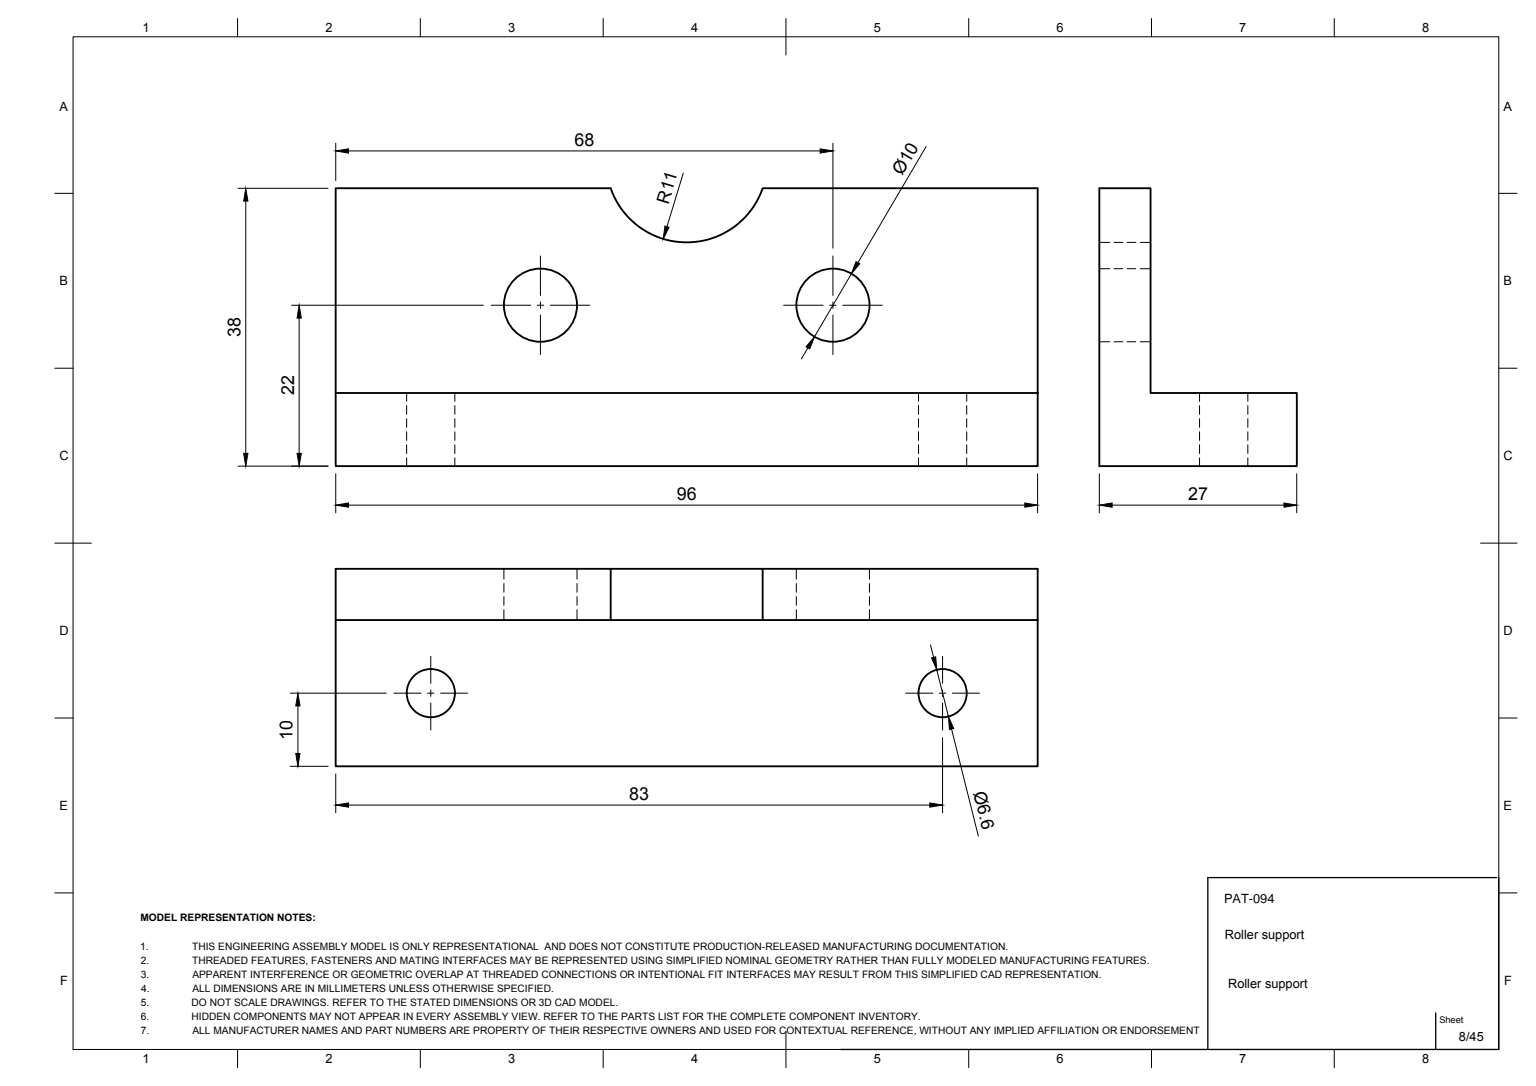
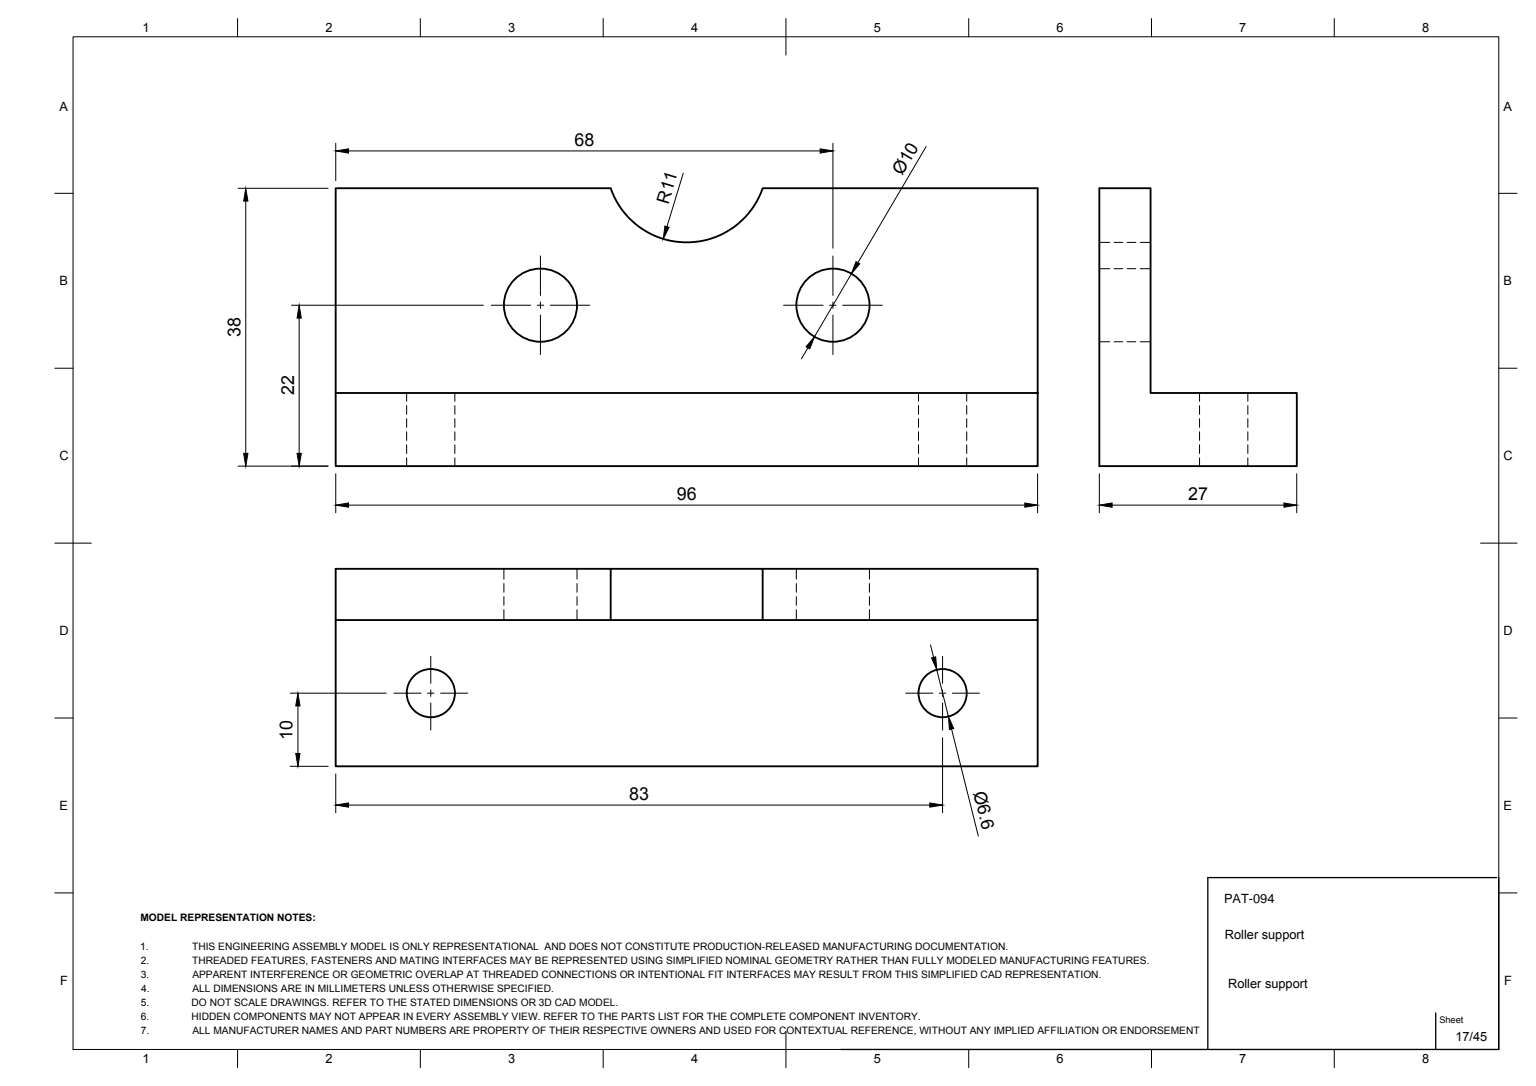
ISO-10303-21;
HEADER;
/* Generated by software containing ST-Developer
 * from STEP Tools, Inc. (www.steptools.com) 
 */

FILE_DESCRIPTION(
/* description */ ('Shaft runout checking stand'),
/* implementation_level */ '2;1');

FILE_NAME(
/* name */ 'Roller support.step',
/* time_stamp */ '2026-11-02T21:12:33-08:00',
/* author */ (''),
/* organization */ (''),
/* preprocessor_version */ 'ST-DEVELOPER v20.2',
/* originating_system */ 'Autodesk Translation Framework v15.17.0.0',
/* authorisation */ '');

FILE_SCHEMA (('AUTOMOTIVE_DESIGN { 1 0 10303 214 3 1 1 }'));
ENDSEC;

DATA;
#10=MECHANICAL_DESIGN_GEOMETRIC_PRESENTATION_REPRESENTATION('',(#469),#11748);
#383=SHAPE_REPRESENTATION_RELATIONSHIP('SRR','None',#11932,#426);
#426=ADVANCED_BREP_SHAPE_REPRESENTATION('',(#520),#11708);
#469=STYLED_ITEM('',(#12169),#520);
#520=MANIFOLD_SOLID_BREP('Body1',#6212);
#591=FACE_BOUND('',#1535,.T.);
#592=FACE_BOUND('',#1536,.T.);
#593=FACE_BOUND('',#1541,.T.);
#594=FACE_BOUND('',#1542,.T.);
#595=FACE_BOUND('',#1546,.T.);
#596=FACE_BOUND('',#1547,.T.);
#597=FACE_BOUND('',#1551,.T.);
#598=FACE_BOUND('',#1552,.T.);
#708=CIRCLE('',#6877,0.33);
#709=CIRCLE('',#6878,0.33);
#710=CIRCLE('',#6880,0.33);
#711=CIRCLE('',#6881,0.33);
#712=CIRCLE('',#6883,1.1);
#713=CIRCLE('',#6884,1.1);
#714=CIRCLE('',#6886,0.5);
#715=CIRCLE('',#6887,0.5);
#716=CIRCLE('',#6890,0.5);
#717=CIRCLE('',#6892,0.5);
#954=CYLINDRICAL_SURFACE('',#6876,0.33);
#955=CYLINDRICAL_SURFACE('',#6879,0.33);
#956=CYLINDRICAL_SURFACE('',#6882,1.1);
#957=CYLINDRICAL_SURFACE('',#6889,0.5);
#958=CYLINDRICAL_SURFACE('',#6891,0.5);
#1134=FACE_OUTER_BOUND('',#1531,.T.);
#1135=FACE_OUTER_BOUND('',#1532,.T.);
#1136=FACE_OUTER_BOUND('',#1533,.T.);
#1137=FACE_OUTER_BOUND('',#1534,.T.);
#1138=FACE_OUTER_BOUND('',#1537,.T.);
#1139=FACE_OUTER_BOUND('',#1538,.T.);
#1140=FACE_OUTER_BOUND('',#1539,.T.);
#1141=FACE_OUTER_BOUND('',#1540,.T.);
#1142=FACE_OUTER_BOUND('',#1543,.T.);
#1143=FACE_OUTER_BOUND('',#1544,.T.);
#1144=FACE_OUTER_BOUND('',#1545,.T.);
#1145=FACE_OUTER_BOUND('',#1548,.T.);
#1146=FACE_OUTER_BOUND('',#1549,.T.);
#1147=FACE_OUTER_BOUND('',#1550,.T.);
#1531=EDGE_LOOP('',(#4596,#4597,#4598,#4599));
#1532=EDGE_LOOP('',(#4600,#4601,#4602,#4603));
#1533=EDGE_LOOP('',(#4604,#4605,#4606,#4607));
#1534=EDGE_LOOP('',(#4608,#4609,#4610,#4611,#4612,#4613));
#1535=EDGE_LOOP('',(#4614));
#1536=EDGE_LOOP('',(#4615));
#1537=EDGE_LOOP('',(#4616,#4617,#4618,#4619));
#1538=EDGE_LOOP('',(#4620,#4621,#4622,#4623));
#1539=EDGE_LOOP('',(#4624,#4625,#4626,#4627));
#1540=EDGE_LOOP('',(#4628,#4629,#4630,#4631));
#1541=EDGE_LOOP('',(#4632));
#1542=EDGE_LOOP('',(#4633));
#1543=EDGE_LOOP('',(#4634,#4635,#4636,#4637));
#1544=EDGE_LOOP('',(#4638,#4639,#4640,#4641,#4642,#4643));
#1545=EDGE_LOOP('',(#4644,#4645,#4646,#4647,#4648,#4649));
#1546=EDGE_LOOP('',(#4650));
#1547=EDGE_LOOP('',(#4651));
#1548=EDGE_LOOP('',(#4652,#4653,#4654,#4655,#4656,#4657));
#1549=EDGE_LOOP('',(#4658,#4659,#4660,#4661));
#1550=EDGE_LOOP('',(#4662,#4663,#4664,#4665));
#1551=EDGE_LOOP('',(#4666));
#1552=EDGE_LOOP('',(#4667));
#2102=LINE('',#10007,#2569);
#2103=LINE('',#10013,#2570);
#2104=LINE('',#10020,#2571);
#2105=LINE('',#10023,#2572);
#2106=LINE('',#10026,#2573);
#2107=LINE('',#10028,#2574);
#2108=LINE('',#10030,#2575);
#2109=LINE('',#10032,#2576);
#2110=LINE('',#10033,#2577);
#2111=LINE('',#10040,#2578);
#2112=LINE('',#10041,#2579);
#2113=LINE('',#10045,#2580);
#2114=LINE('',#10049,#2581);
#2115=LINE('',#10053,#2582);
#2116=LINE('',#10055,#2583);
#2117=LINE('',#10057,#2584);
#2118=LINE('',#10058,#2585);
#2119=LINE('',#10061,#2586);
#2120=LINE('',#10063,#2587);
#2121=LINE('',#10064,#2588);
#2122=LINE('',#10066,#2589);
#2123=LINE('',#10067,#2590);
#2124=LINE('',#10070,#2591);
#2125=LINE('',#10071,#2592);
#2126=LINE('',#10073,#2593);
#2127=LINE('',#10074,#2594);
#2569=VECTOR('',#7997,0.33);
#2570=VECTOR('',#8004,0.33);
#2571=VECTOR('',#8011,1.);
#2572=VECTOR('',#8014,1.);
#2573=VECTOR('',#8017,1.);
#2574=VECTOR('',#8018,1.);
#2575=VECTOR('',#8019,1.);
#2576=VECTOR('',#8020,1.);
#2577=VECTOR('',#8021,1.);
#2578=VECTOR('',#8028,1.);
#2579=VECTOR('',#8029,1.);
#2580=VECTOR('',#8034,0.5);
#2581=VECTOR('',#8039,0.5);
#2582=VECTOR('',#8042,1.);
#2583=VECTOR('',#8043,1.);
#2584=VECTOR('',#8044,1.);
#2585=VECTOR('',#8045,1.);
#2586=VECTOR('',#8048,1.);
#2587=VECTOR('',#8049,1.);
#2588=VECTOR('',#8050,1.);
#2589=VECTOR('',#8053,1.);
#2590=VECTOR('',#8054,1.);
#2591=VECTOR('',#8057,1.);
#2592=VECTOR('',#8058,1.);
#2593=VECTOR('',#8061,1.);
#2594=VECTOR('',#8062,1.);
#2988=VERTEX_POINT('',#10004);
#2989=VERTEX_POINT('',#10006);
#2990=VERTEX_POINT('',#10010);
#2991=VERTEX_POINT('',#10012);
#2992=VERTEX_POINT('',#10016);
#2993=VERTEX_POINT('',#10017);
#2994=VERTEX_POINT('',#10019);
#2995=VERTEX_POINT('',#10021);
#2996=VERTEX_POINT('',#10025);
#2997=VERTEX_POINT('',#10027);
#2998=VERTEX_POINT('',#10029);
#2999=VERTEX_POINT('',#10031);
#3000=VERTEX_POINT('',#10034);
#3001=VERTEX_POINT('',#10036);
#3002=VERTEX_POINT('',#10039);
#3003=VERTEX_POINT('',#10043);
#3004=VERTEX_POINT('',#10047);
#3005=VERTEX_POINT('',#10051);
#3006=VERTEX_POINT('',#10052);
#3007=VERTEX_POINT('',#10054);
#3008=VERTEX_POINT('',#10056);
#3009=VERTEX_POINT('',#10060);
#3010=VERTEX_POINT('',#10062);
#3011=VERTEX_POINT('',#10069);
#3584=EDGE_CURVE('',#2988,#2988,#708,.T.);
#3585=EDGE_CURVE('',#2988,#2989,#2102,.T.);
#3586=EDGE_CURVE('',#2989,#2989,#709,.T.);
#3587=EDGE_CURVE('',#2990,#2990,#710,.T.);
#3588=EDGE_CURVE('',#2990,#2991,#2103,.T.);
#3589=EDGE_CURVE('',#2991,#2991,#711,.T.);
#3590=EDGE_CURVE('',#2992,#2993,#712,.T.);
#3591=EDGE_CURVE('',#2994,#2992,#2104,.T.);
#3592=EDGE_CURVE('',#2995,#2994,#713,.T.);
#3593=EDGE_CURVE('',#2993,#2995,#2105,.T.);
#3594=EDGE_CURVE('',#2996,#2994,#2106,.T.);
#3595=EDGE_CURVE('',#2997,#2996,#2107,.T.);
#3596=EDGE_CURVE('',#2997,#2998,#2108,.T.);
#3597=EDGE_CURVE('',#2998,#2999,#2109,.T.);
#3598=EDGE_CURVE('',#2995,#2999,#2110,.T.);
#3599=EDGE_CURVE('',#3000,#3000,#714,.T.);
#3600=EDGE_CURVE('',#3001,#3001,#715,.T.);
#3601=EDGE_CURVE('',#2992,#3002,#2111,.T.);
#3602=EDGE_CURVE('',#3002,#2996,#2112,.T.);
#3603=EDGE_CURVE('',#3003,#3003,#716,.T.);
#3604=EDGE_CURVE('',#3003,#3001,#2113,.T.);
#3605=EDGE_CURVE('',#3004,#3004,#717,.T.);
#3606=EDGE_CURVE('',#3004,#3000,#2114,.T.);
#3607=EDGE_CURVE('',#3005,#3006,#2115,.T.);
#3608=EDGE_CURVE('',#3005,#3007,#2116,.T.);
#3609=EDGE_CURVE('',#3008,#3007,#2117,.T.);
#3610=EDGE_CURVE('',#3006,#3008,#2118,.T.);
#3611=EDGE_CURVE('',#3006,#3009,#2119,.T.);
#3612=EDGE_CURVE('',#3009,#3010,#2120,.T.);
#3613=EDGE_CURVE('',#3010,#3005,#2121,.T.);
#3614=EDGE_CURVE('',#3010,#2997,#2122,.T.);
#3615=EDGE_CURVE('',#3007,#3002,#2123,.T.);
#3616=EDGE_CURVE('',#3011,#2993,#2124,.T.);
#3617=EDGE_CURVE('',#3008,#3011,#2125,.T.);
#3618=EDGE_CURVE('',#2998,#3009,#2126,.T.);
#3619=EDGE_CURVE('',#2999,#3011,#2127,.T.);
#4596=ORIENTED_EDGE('',*,*,#3584,.F.);
#4597=ORIENTED_EDGE('',*,*,#3585,.T.);
#4598=ORIENTED_EDGE('',*,*,#3586,.F.);
#4599=ORIENTED_EDGE('',*,*,#3585,.F.);
#4600=ORIENTED_EDGE('',*,*,#3587,.F.);
#4601=ORIENTED_EDGE('',*,*,#3588,.T.);
#4602=ORIENTED_EDGE('',*,*,#3589,.F.);
#4603=ORIENTED_EDGE('',*,*,#3588,.F.);
#4604=ORIENTED_EDGE('',*,*,#3590,.F.);
#4605=ORIENTED_EDGE('',*,*,#3591,.F.);
#4606=ORIENTED_EDGE('',*,*,#3592,.F.);
#4607=ORIENTED_EDGE('',*,*,#3593,.F.);
#4608=ORIENTED_EDGE('',*,*,#3592,.T.);
#4609=ORIENTED_EDGE('',*,*,#3594,.F.);
#4610=ORIENTED_EDGE('',*,*,#3595,.F.);
#4611=ORIENTED_EDGE('',*,*,#3596,.T.);
#4612=ORIENTED_EDGE('',*,*,#3597,.T.);
#4613=ORIENTED_EDGE('',*,*,#3598,.F.);
#4614=ORIENTED_EDGE('',*,*,#3599,.T.);
#4615=ORIENTED_EDGE('',*,*,#3600,.T.);
#4616=ORIENTED_EDGE('',*,*,#3591,.T.);
#4617=ORIENTED_EDGE('',*,*,#3601,.T.);
#4618=ORIENTED_EDGE('',*,*,#3602,.T.);
#4619=ORIENTED_EDGE('',*,*,#3594,.T.);
#4620=ORIENTED_EDGE('',*,*,#3603,.F.);
#4621=ORIENTED_EDGE('',*,*,#3604,.T.);
#4622=ORIENTED_EDGE('',*,*,#3600,.F.);
#4623=ORIENTED_EDGE('',*,*,#3604,.F.);
#4624=ORIENTED_EDGE('',*,*,#3605,.F.);
#4625=ORIENTED_EDGE('',*,*,#3606,.T.);
#4626=ORIENTED_EDGE('',*,*,#3599,.F.);
#4627=ORIENTED_EDGE('',*,*,#3606,.F.);
#4628=ORIENTED_EDGE('',*,*,#3607,.F.);
#4629=ORIENTED_EDGE('',*,*,#3608,.T.);
#4630=ORIENTED_EDGE('',*,*,#3609,.F.);
#4631=ORIENTED_EDGE('',*,*,#3610,.F.);
#4632=ORIENTED_EDGE('',*,*,#3586,.T.);
#4633=ORIENTED_EDGE('',*,*,#3589,.T.);
#4634=ORIENTED_EDGE('',*,*,#3607,.T.);
#4635=ORIENTED_EDGE('',*,*,#3611,.T.);
#4636=ORIENTED_EDGE('',*,*,#3612,.T.);
#4637=ORIENTED_EDGE('',*,*,#3613,.T.);
#4638=ORIENTED_EDGE('',*,*,#3614,.T.);
#4639=ORIENTED_EDGE('',*,*,#3595,.T.);
#4640=ORIENTED_EDGE('',*,*,#3602,.F.);
#4641=ORIENTED_EDGE('',*,*,#3615,.F.);
#4642=ORIENTED_EDGE('',*,*,#3608,.F.);
#4643=ORIENTED_EDGE('',*,*,#3613,.F.);
#4644=ORIENTED_EDGE('',*,*,#3590,.T.);
#4645=ORIENTED_EDGE('',*,*,#3616,.F.);
#4646=ORIENTED_EDGE('',*,*,#3617,.F.);
#4647=ORIENTED_EDGE('',*,*,#3609,.T.);
#4648=ORIENTED_EDGE('',*,*,#3615,.T.);
#4649=ORIENTED_EDGE('',*,*,#3601,.F.);
#4650=ORIENTED_EDGE('',*,*,#3603,.T.);
#4651=ORIENTED_EDGE('',*,*,#3605,.T.);
#4652=ORIENTED_EDGE('',*,*,#3618,.T.);
#4653=ORIENTED_EDGE('',*,*,#3611,.F.);
#4654=ORIENTED_EDGE('',*,*,#3610,.T.);
#4655=ORIENTED_EDGE('',*,*,#3617,.T.);
#4656=ORIENTED_EDGE('',*,*,#3619,.F.);
#4657=ORIENTED_EDGE('',*,*,#3597,.F.);
#4658=ORIENTED_EDGE('',*,*,#3593,.T.);
#4659=ORIENTED_EDGE('',*,*,#3598,.T.);
#4660=ORIENTED_EDGE('',*,*,#3619,.T.);
#4661=ORIENTED_EDGE('',*,*,#3616,.T.);
#4662=ORIENTED_EDGE('',*,*,#3618,.F.);
#4663=ORIENTED_EDGE('',*,*,#3596,.F.);
#4664=ORIENTED_EDGE('',*,*,#3614,.F.);
#4665=ORIENTED_EDGE('',*,*,#3612,.F.);
#4666=ORIENTED_EDGE('',*,*,#3584,.T.);
#4667=ORIENTED_EDGE('',*,*,#3587,.T.);
#5683=PLANE('',#6885);
#5684=PLANE('',#6888);
#5685=PLANE('',#6893);
#5686=PLANE('',#6894);
#5687=PLANE('',#6895);
#5688=PLANE('',#6896);
#5689=PLANE('',#6897);
#5690=PLANE('',#6898);
#5691=PLANE('',#6899);
#5934=ADVANCED_FACE('',(#1134),#954,.F.);
#5935=ADVANCED_FACE('',(#1135),#955,.F.);
#5936=ADVANCED_FACE('',(#1136),#956,.F.);
#5937=ADVANCED_FACE('',(#1137,#591,#592),#5683,.T.);
#5938=ADVANCED_FACE('',(#1138),#5684,.T.);
#5939=ADVANCED_FACE('',(#1139),#957,.F.);
#5940=ADVANCED_FACE('',(#1140),#958,.F.);
#5941=ADVANCED_FACE('',(#1141,#593,#594),#5685,.T.);
#5942=ADVANCED_FACE('',(#1142),#5686,.F.);
#5943=ADVANCED_FACE('',(#1143),#5687,.T.);
#5944=ADVANCED_FACE('',(#1144,#595,#596),#5688,.T.);
#5945=ADVANCED_FACE('',(#1145),#5689,.T.);
#5946=ADVANCED_FACE('',(#1146),#5690,.T.);
#5947=ADVANCED_FACE('',(#1147,#597,#598),#5691,.F.);
#6212=CLOSED_SHELL('',(#5934,#5935,#5936,#5937,#5938,#5939,#5940,#5941,
#5942,#5943,#5944,#5945,#5946,#5947));
#6875=AXIS2_PLACEMENT_3D('',#10002,#7991,#7992);
#6876=AXIS2_PLACEMENT_3D('',#10003,#7993,#7994);
#6877=AXIS2_PLACEMENT_3D('',#10005,#7995,#7996);
#6878=AXIS2_PLACEMENT_3D('',#10008,#7998,#7999);
#6879=AXIS2_PLACEMENT_3D('',#10009,#8000,#8001);
#6880=AXIS2_PLACEMENT_3D('',#10011,#8002,#8003);
#6881=AXIS2_PLACEMENT_3D('',#10014,#8005,#8006);
#6882=AXIS2_PLACEMENT_3D('',#10015,#8007,#8008);
#6883=AXIS2_PLACEMENT_3D('',#10018,#8009,#8010);
#6884=AXIS2_PLACEMENT_3D('',#10022,#8012,#8013);
#6885=AXIS2_PLACEMENT_3D('',#10024,#8015,#8016);
#6886=AXIS2_PLACEMENT_3D('',#10035,#8022,#8023);
#6887=AXIS2_PLACEMENT_3D('',#10037,#8024,#8025);
#6888=AXIS2_PLACEMENT_3D('',#10038,#8026,#8027);
#6889=AXIS2_PLACEMENT_3D('',#10042,#8030,#8031);
#6890=AXIS2_PLACEMENT_3D('',#10044,#8032,#8033);
#6891=AXIS2_PLACEMENT_3D('',#10046,#8035,#8036);
#6892=AXIS2_PLACEMENT_3D('',#10048,#8037,#8038);
#6893=AXIS2_PLACEMENT_3D('',#10050,#8040,#8041);
#6894=AXIS2_PLACEMENT_3D('',#10059,#8046,#8047);
#6895=AXIS2_PLACEMENT_3D('',#10065,#8051,#8052);
#6896=AXIS2_PLACEMENT_3D('',#10068,#8055,#8056);
#6897=AXIS2_PLACEMENT_3D('',#10072,#8059,#8060);
#6898=AXIS2_PLACEMENT_3D('',#10075,#8063,#8064);
#6899=AXIS2_PLACEMENT_3D('',#10076,#8065,#8066);
#7991=DIRECTION('axis',(0.,0.,1.));
#7992=DIRECTION('refdir',(1.,0.,0.));
#7993=DIRECTION('center_axis',(0.,0.,1.));
#7994=DIRECTION('ref_axis',(1.,0.,0.));
#7995=DIRECTION('center_axis',(0.,0.,1.));
#7996=DIRECTION('ref_axis',(1.,0.,0.));
#7997=DIRECTION('',(0.,0.,1.));
#7998=DIRECTION('center_axis',(0.,0.,-1.));
#7999=DIRECTION('ref_axis',(1.,0.,0.));
#8000=DIRECTION('center_axis',(0.,0.,1.));
#8001=DIRECTION('ref_axis',(1.,0.,0.));
#8002=DIRECTION('center_axis',(0.,0.,1.));
#8003=DIRECTION('ref_axis',(1.,0.,0.));
#8004=DIRECTION('',(0.,0.,1.));
#8005=DIRECTION('center_axis',(0.,0.,-1.));
#8006=DIRECTION('ref_axis',(1.,0.,0.));
#8007=DIRECTION('center_axis',(0.,1.,0.));
#8008=DIRECTION('ref_axis',(1.,0.,0.));
#8009=DIRECTION('center_axis',(0.,1.,0.));
#8010=DIRECTION('ref_axis',(1.,0.,0.));
#8011=DIRECTION('',(0.,-1.,0.));
#8012=DIRECTION('center_axis',(0.,-1.,0.));
#8013=DIRECTION('ref_axis',(1.,0.,0.));
#8014=DIRECTION('',(0.,1.,0.));
#8015=DIRECTION('center_axis',(0.,1.,0.));
#8016=DIRECTION('ref_axis',(-1.,0.,0.));
#8017=DIRECTION('',(-1.,0.,0.));
#8018=DIRECTION('',(0.,0.,1.));
#8019=DIRECTION('',(-1.,0.,0.));
#8020=DIRECTION('',(0.,0.,1.));
#8021=DIRECTION('',(-1.,0.,0.));
#8022=DIRECTION('center_axis',(0.,-1.,0.));
#8023=DIRECTION('ref_axis',(1.,0.,0.));
#8024=DIRECTION('center_axis',(0.,-1.,0.));
#8025=DIRECTION('ref_axis',(1.,0.,0.));
#8026=DIRECTION('center_axis',(0.,0.,1.));
#8027=DIRECTION('ref_axis',(1.,0.,0.));
#8028=DIRECTION('',(1.,0.,0.));
#8029=DIRECTION('',(0.,1.,0.));
#8030=DIRECTION('center_axis',(0.,1.,0.));
#8031=DIRECTION('ref_axis',(1.,0.,0.));
#8032=DIRECTION('center_axis',(0.,1.,0.));
#8033=DIRECTION('ref_axis',(1.,0.,0.));
#8034=DIRECTION('',(0.,1.,0.));
#8035=DIRECTION('center_axis',(0.,1.,0.));
#8036=DIRECTION('ref_axis',(1.,0.,0.));
#8037=DIRECTION('center_axis',(0.,1.,0.));
#8038=DIRECTION('ref_axis',(1.,0.,0.));
#8039=DIRECTION('',(0.,1.,0.));
#8040=DIRECTION('center_axis',(0.,0.,1.));
#8041=DIRECTION('ref_axis',(1.,0.,0.));
#8042=DIRECTION('',(-1.,0.,0.));
#8043=DIRECTION('',(0.,1.,0.));
#8044=DIRECTION('',(1.,0.,0.));
#8045=DIRECTION('',(0.,1.,0.));
#8046=DIRECTION('center_axis',(0.,1.,0.));
#8047=DIRECTION('ref_axis',(1.,0.,0.));
#8048=DIRECTION('',(0.,0.,-1.));
#8049=DIRECTION('',(1.,0.,0.));
#8050=DIRECTION('',(0.,0.,1.));
#8051=DIRECTION('center_axis',(1.,0.,0.));
#8052=DIRECTION('ref_axis',(0.,1.,0.));
#8053=DIRECTION('',(0.,1.,0.));
#8054=DIRECTION('',(0.,0.,1.));
#8055=DIRECTION('center_axis',(0.,-1.,0.));
#8056=DIRECTION('ref_axis',(1.,0.,0.));
#8057=DIRECTION('',(1.,0.,0.));
#8058=DIRECTION('',(0.,0.,1.));
#8059=DIRECTION('center_axis',(-1.,0.,0.));
#8060=DIRECTION('ref_axis',(0.,-1.,0.));
#8061=DIRECTION('',(0.,-1.,0.));
#8062=DIRECTION('',(0.,-1.,0.));
#8063=DIRECTION('center_axis',(0.,0.,1.));
#8064=DIRECTION('ref_axis',(1.,0.,0.));
#8065=DIRECTION('center_axis',(0.,0.,1.));
#8066=DIRECTION('ref_axis',(1.,0.,0.));
#10002=CARTESIAN_POINT('',(0.,0.,0.));
#10003=CARTESIAN_POINT('Origin',(-3.5,-12.5,2.7));
#10004=CARTESIAN_POINT('',(-3.83,-12.5,2.8));
#10005=CARTESIAN_POINT('Origin',(-3.5,-12.5,2.8));
#10006=CARTESIAN_POINT('',(-3.83,-12.5,3.8));
#10007=CARTESIAN_POINT('',(-3.83,-12.5,2.7));
#10008=CARTESIAN_POINT('Origin',(-3.5,-12.5,3.8));
#10009=CARTESIAN_POINT('Origin',(3.5,-12.5,2.7));
#10010=CARTESIAN_POINT('',(3.17,-12.5,2.8));
#10011=CARTESIAN_POINT('Origin',(3.5,-12.5,2.8));
#10012=CARTESIAN_POINT('',(3.17,-12.5,3.8));
#10013=CARTESIAN_POINT('',(3.17,-12.5,2.7));
#10014=CARTESIAN_POINT('Origin',(3.5,-12.5,3.8));
#10015=CARTESIAN_POINT('Origin',(0.,-11.6,6.95959179422654));
#10016=CARTESIAN_POINT('',(1.03956420750473,-11.5,6.6));
#10017=CARTESIAN_POINT('',(-1.03956420750473,-11.5,6.6));
#10018=CARTESIAN_POINT('Origin',(0.,-11.5,6.95959179422654));
#10019=CARTESIAN_POINT('',(1.03956420750473,-10.8,6.6));
#10020=CARTESIAN_POINT('',(1.03956420750473,-11.6,6.6));
#10021=CARTESIAN_POINT('',(-1.03956420750473,-10.8,6.6));
#10022=CARTESIAN_POINT('Origin',(0.,-10.8,6.95959179422654));
#10023=CARTESIAN_POINT('',(-1.03956420750473,-11.6,6.6));
#10024=CARTESIAN_POINT('Origin',(4.8,-10.8,2.8));
#10025=CARTESIAN_POINT('',(4.8,-10.8,6.6));
#10026=CARTESIAN_POINT('',(4.8,-10.8,6.6));
#10027=CARTESIAN_POINT('',(4.8,-10.8,2.8));
#10028=CARTESIAN_POINT('',(4.8,-10.8,2.8));
#10029=CARTESIAN_POINT('',(-4.8,-10.8,2.8));
#10030=CARTESIAN_POINT('',(4.8,-10.8,2.8));
#10031=CARTESIAN_POINT('',(-4.8,-10.8,6.6));
#10032=CARTESIAN_POINT('',(-4.8,-10.8,2.8));
#10033=CARTESIAN_POINT('',(4.8,-10.8,6.6));
#10034=CARTESIAN_POINT('',(1.5,-10.8,5.));
#10035=CARTESIAN_POINT('Origin',(2.,-10.8,5.));
#10036=CARTESIAN_POINT('',(-2.5,-10.8,5.));
#10037=CARTESIAN_POINT('Origin',(-2.,-10.8,5.));
#10038=CARTESIAN_POINT('Origin',(0.,-11.15,6.6));
#10039=CARTESIAN_POINT('',(4.8,-11.5,6.6));
#10040=CARTESIAN_POINT('',(-4.8,-11.5,6.6));
#10041=CARTESIAN_POINT('',(4.8,-11.5,6.6));
#10042=CARTESIAN_POINT('Origin',(-2.,-11.6,5.));
#10043=CARTESIAN_POINT('',(-2.5,-11.5,5.));
#10044=CARTESIAN_POINT('Origin',(-2.,-11.5,5.));
#10045=CARTESIAN_POINT('',(-2.5,-11.6,5.));
#10046=CARTESIAN_POINT('Origin',(2.,-11.6,5.));
#10047=CARTESIAN_POINT('',(1.5,-11.5,5.));
#10048=CARTESIAN_POINT('Origin',(2.,-11.5,5.));
#10049=CARTESIAN_POINT('',(1.5,-11.6,5.));
#10050=CARTESIAN_POINT('Origin',(-4.8,-13.5,3.8));
#10051=CARTESIAN_POINT('',(4.8,-13.5,3.8));
#10052=CARTESIAN_POINT('',(-4.8,-13.5,3.8));
#10053=CARTESIAN_POINT('',(4.8,-13.5,3.8));
#10054=CARTESIAN_POINT('',(4.8,-11.5,3.8));
#10055=CARTESIAN_POINT('',(4.8,-13.5,3.8));
#10056=CARTESIAN_POINT('',(-4.8,-11.5,3.8));
#10057=CARTESIAN_POINT('',(-4.8,-11.5,3.8));
#10058=CARTESIAN_POINT('',(-4.8,-13.5,3.8));
#10059=CARTESIAN_POINT('Origin',(0.,-13.5,3.3));
#10060=CARTESIAN_POINT('',(-4.8,-13.5,2.8));
#10061=CARTESIAN_POINT('',(-4.8,-13.5,3.8));
#10062=CARTESIAN_POINT('',(4.8,-13.5,2.8));
#10063=CARTESIAN_POINT('',(-4.8,-13.5,2.8));
#10064=CARTESIAN_POINT('',(4.8,-13.5,2.8));
#10065=CARTESIAN_POINT('Origin',(4.8,-11.5,2.8));
#10066=CARTESIAN_POINT('',(4.8,-13.5,2.8));
#10067=CARTESIAN_POINT('',(4.8,-11.5,2.8));
#10068=CARTESIAN_POINT('Origin',(-4.8,-11.5,2.8));
#10069=CARTESIAN_POINT('',(-4.8,-11.5,6.6));
#10070=CARTESIAN_POINT('',(-4.8,-11.5,6.6));
#10071=CARTESIAN_POINT('',(-4.8,-11.5,2.8));
#10072=CARTESIAN_POINT('Origin',(-4.8,-10.8,2.8));
#10073=CARTESIAN_POINT('',(-4.8,-10.8,2.8));
#10074=CARTESIAN_POINT('',(-4.8,-10.8,6.6));
#10075=CARTESIAN_POINT('Origin',(0.,-11.15,6.6));
#10076=CARTESIAN_POINT('Origin',(0.,-11.15,2.8));
#11659=UNCERTAINTY_MEASURE_WITH_UNIT(LENGTH_MEASURE(0.001),#11749,
'DISTANCE_ACCURACY_VALUE',
'Maximum model space distance between geometric entities at asserted c
onnectivities');
#11699=UNCERTAINTY_MEASURE_WITH_UNIT(LENGTH_MEASURE(0.001),#11749,
'DISTANCE_ACCURACY_VALUE',
'Maximum model space distance between geometric entities at asserted c
onnectivities');
#11708=(
GEOMETRIC_REPRESENTATION_CONTEXT(3)
GLOBAL_UNCERTAINTY_ASSIGNED_CONTEXT((#11659))
GLOBAL_UNIT_ASSIGNED_CONTEXT((#11749,#11751,#11752))
REPRESENTATION_CONTEXT('','3D')
);
#11748=(
GEOMETRIC_REPRESENTATION_CONTEXT(3)
GLOBAL_UNCERTAINTY_ASSIGNED_CONTEXT((#11699))
GLOBAL_UNIT_ASSIGNED_CONTEXT((#11749,#11751,#11752))
REPRESENTATION_CONTEXT('','3D')
);
#11749=(
LENGTH_UNIT()
NAMED_UNIT(*)
SI_UNIT(.CENTI.,.METRE.)
);
#11751=(
NAMED_UNIT(*)
PLANE_ANGLE_UNIT()
SI_UNIT($,.RADIAN.)
);
#11752=(
NAMED_UNIT(*)
SI_UNIT($,.STERADIAN.)
SOLID_ANGLE_UNIT()
);
#11761=SHAPE_DEFINITION_REPRESENTATION(#11809,#11932);
#11809=PRODUCT_DEFINITION_SHAPE('',$,#11981);
#11932=SHAPE_REPRESENTATION('',(#6875),#11708);
#11972=PRODUCT_DEFINITION_CONTEXT('part definition',#12118,'design');
#11981=PRODUCT_DEFINITION('Roller support','Roller support',#12029,#11972);
#12029=PRODUCT_DEFINITION_FORMATION('',$,#12128);
#12118=APPLICATION_CONTEXT(
'Core Data for Automotive Mechanical Design Process');
#12119=PRODUCT_CONTEXT('part definition',#12118,'mechanical');
#12128=PRODUCT('Roller support','Roller support','Roller support',(#12119));
#12169=PRESENTATION_STYLE_ASSIGNMENT((#12174));
#12174=SURFACE_STYLE_USAGE(.BOTH.,#12179);
#12179=SURFACE_SIDE_STYLE('',(#12184));
#12184=SURFACE_STYLE_FILL_AREA(#12189);
#12189=FILL_AREA_STYLE('CAD Library Painted - Engineering blue',(#12194));
#12194=FILL_AREA_STYLE_COLOUR('CAD Library Painted - Engineering blue',
#12199);
#12199=COLOUR_RGB('CAD Library Painted - Engineering blue',0.12156862745098,
0.356862745098039,0.6);
ENDSEC;
END-ISO-10303-21;
